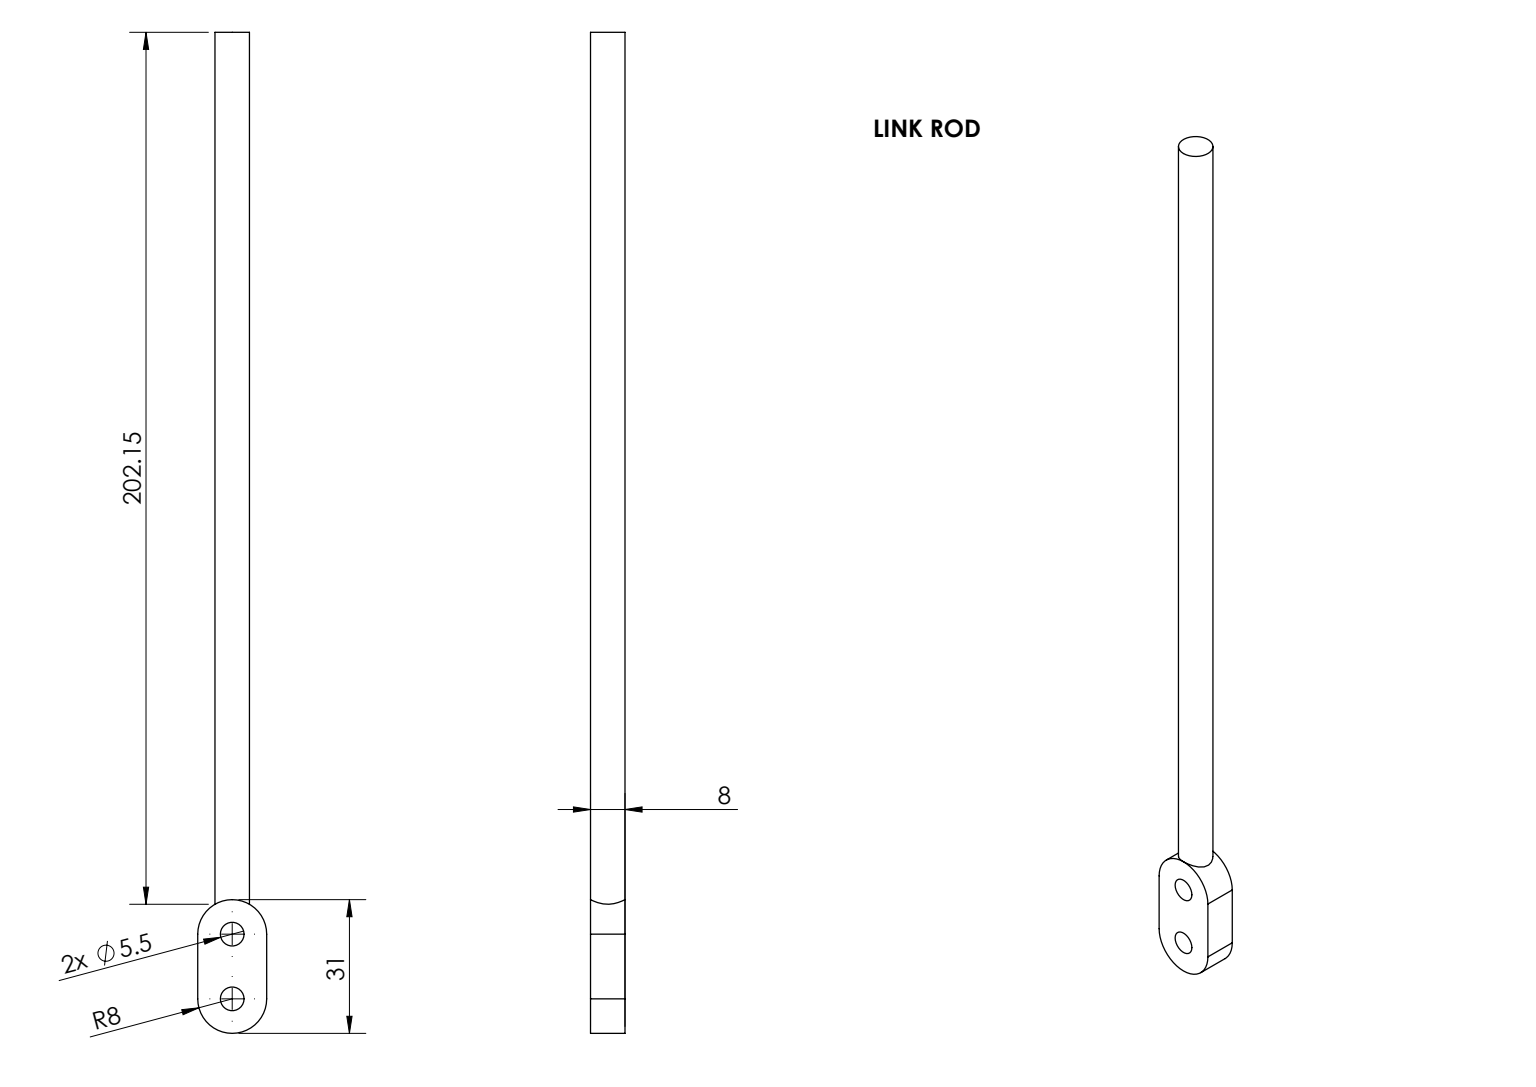
ISO-10303-21;
HEADER;
FILE_DESCRIPTION (('STEP AP214'),
    '1' );
FILE_NAME ('link rod.step',
    '2026-09-24T10:26:00',
    ( '' ),
    ( '' ),
    'SwSTEP 2.0',
    'SolidWorks 2026',
    '' );
FILE_SCHEMA (( 'AUTOMOTIVE_DESIGN' ));
ENDSEC;

DATA;
#140=DIRECTION ( 'NONE',  ( 0.000000000000000000, 1.000000000000000000, 0.000000000000000000 ) ) ;
#167=CARTESIAN_POINT ( 'NONE',  ( 0.000000000000000000, 0.000000000000000000, 0.000000000000000000 ) ) ;
#178=LINE ( 'NONE', #1338, #11397 ) ;
#188=AXIS2_PLACEMENT_3D ( 'NONE', #12778, #9636, #495 ) ;
#201=VECTOR ( 'NONE', #12349, 1000.000000000000000 ) ;
#214=CARTESIAN_POINT ( 'NONE',  ( 8.000000000000000000, 25.49999999999996803, 8.000000000000007105 ) ) ;
#231=FILL_AREA_STYLE_COLOUR ( '', #8450 ) ;
#235=CARTESIAN_POINT ( 'NONE',  ( 0.000000000000000000, 25.49999999999996803, 8.000000000000007105 ) ) ;
#292=ORIENTED_EDGE ( 'NONE', *, *, #11801, .F. ) ;
#308=AXIS2_PLACEMENT_3D ( 'NONE', #4405, #11111, #14418 ) ;
#313=VERTEX_POINT ( 'NONE', #3807 ) ;
#351=DIRECTION ( 'NONE',  ( 0.000000000000000000, 0.000000000000000000, 1.000000000000000000 ) ) ;
#354=CARTESIAN_POINT ( 'NONE',  ( -2.749999999999997780, 25.49999999999996803, 8.000000000000007105 ) ) ;
#363=FACE_BOUND ( 'NONE', #5930, .T. ) ;
#377=ADVANCED_FACE ( 'NONE', ( #4324 ), #12061, .F. ) ;
#423=VECTOR ( 'NONE', #878, 1000.000000000000000 ) ;
#495=DIRECTION ( 'NONE',  ( 1.000000000000000000, 0.000000000000000000, 0.000000000000000000 ) ) ;
#501=DIRECTION ( 'NONE',  ( 0.000000000000000000, 0.000000000000000000, -1.000000000000000000 ) ) ;
#504=EDGE_LOOP ( 'NONE', ( #9711, #6187, #8657, #5376, #2686 ) ) ;
#531=FACE_OUTER_BOUND ( 'NONE', #7015, .T. ) ;
#549=VERTEX_POINT ( 'NONE', #5876 ) ;
#557=ADVANCED_FACE ( 'NONE', ( #2536 ), #12548, .F. ) ;
#617=ORIENTED_EDGE ( 'NONE', *, *, #13492, .F. ) ;
#662=EDGE_CURVE ( 'NONE', #4679, #9332, #11674, .T. ) ;
#667=CARTESIAN_POINT ( 'NONE',  ( 2.450325270861126281, 48.11882021490242778, 7.172319002129951215 ) ) ;
#827=AXIS2_PLACEMENT_3D ( 'NONE', #1064, #4522, #2445 ) ;
#840=CARTESIAN_POINT ( 'NONE',  ( -3.010143253645307659, 47.91462539009204136, 1.353322078536347339 ) ) ;
#846=DIRECTION ( 'NONE',  ( 0.000000000000000000, 0.000000000000000000, 1.000000000000000000 ) ) ;
#859=CARTESIAN_POINT ( 'NONE',  ( 3.466359554492712824, 47.71176265719417131, 6.012830585829956220 ) ) ;
#878=DIRECTION ( 'NONE',  ( 0.000000000000000000, 1.000000000000000000, 0.000000000000000000 ) ) ;
#886=EDGE_CURVE ( 'NONE', #11486, #7236, #4159, .T. ) ;
#927=CARTESIAN_POINT ( 'NONE',  ( 3.973244831464914029, 47.44383994248515535, 3.467973375954350512 ) ) ;
#978=VECTOR ( 'NONE', #140, 1000.000000000000000 ) ;
#1006=LINE ( 'NONE', #1078, #7921 ) ;
#1010=LINE ( 'NONE', #4471, #7742 ) ;
#1036=EDGE_LOOP ( 'NONE', ( #12151, #2448, #6023, #13812 ) ) ;
#1048=CARTESIAN_POINT ( 'NONE',  ( 2.750000000000003553, 40.49999999999999289, 8.000000000000007105 ) ) ;
#1064=CARTESIAN_POINT ( 'NONE',  ( 0.000000000000000000, 40.49999999999999289, 8.000000000000007105 ) ) ;
#1078=CARTESIAN_POINT ( 'NONE',  ( -8.000000000000000000, 40.49999999999999289, 8.000000000000007105 ) ) ;
#1113=DIRECTION ( 'NONE',  ( 0.000000000000000000, 0.000000000000000000, 1.000000000000000000 ) ) ;
#1200=( GEOMETRIC_REPRESENTATION_CONTEXT ( 3 ) GLOBAL_UNCERTAINTY_ASSIGNED_CONTEXT ( ( #2815 ) ) GLOBAL_UNIT_ASSIGNED_CONTEXT ( ( #12457, #5770, #9006 ) ) REPRESENTATION_CONTEXT ( 'NONE', 'WORKASPACE' ) );
#1227=CARTESIAN_POINT ( 'NONE',  ( 0.000000000000000000, 17.49899999999995970, 4.000000000000003553 ) ) ;
#1240=CARTESIAN_POINT ( 'NONE',  ( -2.749999999999997780, 25.49999999999996803, 8.000000000000007105 ) ) ;
#1247=DIRECTION ( 'NONE',  ( 0.000000000000000000, 0.000000000000000000, 1.000000000000000000 ) ) ;
#1257=VERTEX_POINT ( 'NONE', #4208 ) ;
#1297=EDGE_CURVE ( 'NONE', #1257, #9332, #10297, .T. ) ;
#1338=CARTESIAN_POINT ( 'NONE',  ( 0.000000000000000000, 17.49899999999995970, 8.000000000000003553 ) ) ;
#1374=LINE ( 'NONE', #9204, #8230 ) ;
#1387=EDGE_CURVE ( 'NONE', #5595, #313, #12174, .T. ) ;
#1395=CYLINDRICAL_SURFACE ( 'NONE', #5325, 8.000000000000000000 ) ;
#1422=EDGE_LOOP ( 'NONE', ( #3931, #617 ) ) ;
#1441=CARTESIAN_POINT ( 'NONE',  ( 0.000000000000000000, 40.49999999999999289, 8.000000000000007105 ) ) ;
#1465=CIRCLE ( 'NONE', #308, 2.749999999999997780 ) ;
#1511=CARTESIAN_POINT ( 'NONE',  ( -2.450325270861127613, 48.11882021490243488, 7.172319002129952992 ) ) ;
#1547=ORIENTED_EDGE ( 'NONE', *, *, #6614, .T. ) ;
#1572=EDGE_LOOP ( 'NONE', ( #7051, #8246 ) ) ;
#1581=FACE_OUTER_BOUND ( 'NONE', #504, .T. ) ;
#1592=ORIENTED_EDGE ( 'NONE', *, *, #11567, .F. ) ;
#1613=FACE_OUTER_BOUND ( 'NONE', #5829, .T. ) ;
#1622=ADVANCED_FACE ( 'NONE', ( #7977 ), #11348, .T. ) ;
#1656=EDGE_LOOP ( 'NONE', ( #4322, #4081, #13598, #12074 ) ) ;
#1691=ADVANCED_FACE ( 'NONE', ( #13566 ), #3537, .F. ) ;
#1693=VERTEX_POINT ( 'NONE', #6222 ) ;
#1714=ORIENTED_EDGE ( 'NONE', *, *, #6615, .T. ) ;
#1724=DIRECTION ( 'NONE',  ( 0.000000000000000000, 0.000000000000000000, 1.000000000000000000 ) ) ;
#1757=CARTESIAN_POINT ( 'NONE',  ( 1.051966859446179514, 48.43488408057972805, 0.1316037626694079310 ) ) ;
#1770=CIRCLE ( 'NONE', #11106, 2.750000000000003553 ) ;
#1805=CARTESIAN_POINT ( 'NONE',  ( -3.466359554492713269, 47.71176265719419973, 6.012830585829961549 ) ) ;
#1825=ADVANCED_FACE ( 'NONE', ( #531 ), #9525, .T. ) ;
#1837=VECTOR ( 'NONE', #8930, 1000.000000000000000 ) ;
#1857=VERTEX_POINT ( 'NONE', #13124 ) ;
#1893=DIRECTION ( 'NONE',  ( 0.000000000000000000, 0.000000000000000000, -1.000000000000000000 ) ) ;
#1912=CIRCLE ( 'NONE', #11248, 8.000000000000000000 ) ;
#1969=ORIENTED_EDGE ( 'NONE', *, *, #4883, .F. ) ;
#1998=CARTESIAN_POINT ( 'NONE',  ( 0.000000000000000000, 48.49999999999999289, 0.000000000000000000 ) ) ;
#2053=DIRECTION ( 'NONE',  ( 0.000000000000000000, 0.000000000000000000, -1.000000000000000000 ) ) ;
#2106=CARTESIAN_POINT ( 'NONE',  ( 0.000000000000000000, 40.49999999999999289, 8.000000000000007105 ) ) ;
#2140=CARTESIAN_POINT ( 'NONE',  ( 8.000000000000000000, 25.49999999999996803, 0.000000000000000000 ) ) ;
#2148=FACE_OUTER_BOUND ( 'NONE', #13063, .T. ) ;
#2189=CARTESIAN_POINT ( 'NONE',  ( 0.000000000000000000, 249.5765550933606391, 8.000000000000003553 ) ) ;
#2229=EDGE_LOOP ( 'NONE', ( #1714, #13927, #11939, #1969 ) ) ;
#2260=DIRECTION ( 'NONE',  ( 0.000000000000000000, 0.000000000000000000, 1.000000000000000000 ) ) ;
#2284=EDGE_CURVE ( 'NONE', #6358, #9561, #1006, .T. ) ;
#2333=AXIS2_PLACEMENT_3D ( 'NONE', #14004, #2053, #4343 ) ;
#2411=EDGE_CURVE ( 'NONE', #6243, #549, #10151, .T. ) ;
#2426=VECTOR ( 'NONE', #5088, 1000.000000000000000 ) ;
#2430=SURFACE_SIDE_STYLE ('',( #5840 ) ) ;
#2445=DIRECTION ( 'NONE',  ( 1.000000000000000000, 0.000000000000000000, 0.000000000000000000 ) ) ;
#2448=ORIENTED_EDGE ( 'NONE', *, *, #6615, .F. ) ;
#2536=FACE_OUTER_BOUND ( 'NONE', #12567, .T. ) ;
#2583=ORIENTED_EDGE ( 'NONE', *, *, #2706, .T. ) ;
#2686=ORIENTED_EDGE ( 'NONE', *, *, #11415, .T. ) ;
#2706=EDGE_CURVE ( 'NONE', #4722, #12253, #4867, .T. ) ;
#2789=AXIS2_PLACEMENT_3D ( 'NONE', #8599, #3200, #3065 ) ;
#2791=CARTESIAN_POINT ( 'NONE',  ( 8.000000000000000000, 40.49999999999999289, 8.000000000000007105 ) ) ;
#2802=CIRCLE ( 'NONE', #9799, 2.750000000000003553 ) ;
#2815=UNCERTAINTY_MEASURE_WITH_UNIT (LENGTH_MEASURE( 1.000000000000000082E-05 ), #12457, 'distance_accuracy_value', 'NONE');
#2866=DIRECTION ( 'NONE',  ( 1.000000000000000000, 0.000000000000000000, 0.000000000000000000 ) ) ;
#2908=EDGE_CURVE ( 'NONE', #313, #5595, #8361, .T. ) ;
#2927=PRESENTATION_STYLE_ASSIGNMENT (( #10808 ) ) ;
#2941=CARTESIAN_POINT ( 'NONE',  ( 1.305984381679704098, 48.39647413643795204, 0.2102513847387766921 ) ) ;
#2988=CARTESIAN_POINT ( 'NONE',  ( -3.012791009409888865, 47.91354231080889292, 6.643648411893776640 ) ) ;
#2993=FILL_AREA_STYLE ('',( #6260 ) ) ;
#3013=CARTESIAN_POINT ( 'NONE',  ( 2.647226096189656985, 48.05180945724377750, 0.9903388192220060615 ) ) ;
#3018=CARTESIAN_POINT ( 'NONE',  ( 0.000000000000000000, 25.49999999999996803, 8.000000000000007105 ) ) ;
#3038=EDGE_LOOP ( 'NONE', ( #1547, #11800, #11167, #13440 ) ) ;
#3065=DIRECTION ( 'NONE',  ( 1.000000000000000000, 0.000000000000000000, 0.000000000000000000 ) ) ;
#3070=DIRECTION ( 'NONE',  ( 0.000000000000000000, 0.000000000000000000, 1.000000000000000000 ) ) ;
#3095=ADVANCED_FACE ( 'NONE', ( #13196 ), #7597, .T. ) ;
#3152=CARTESIAN_POINT ( 'NONE',  ( 3.973178806327566370, 47.44387873568884118, 4.532639216498019152 ) ) ;
#3178=CARTESIAN_POINT ( 'NONE',  ( 8.000000000000000000, 25.49999999999996803, 8.000000000000007105 ) ) ;
#3200=DIRECTION ( 'NONE',  ( 0.000000000000000000, 0.000000000000000000, 1.000000000000000000 ) ) ;
#3216=CARTESIAN_POINT ( 'NONE',  ( 3.010143253645308992, 47.91462539009204136, 1.353322078536349338 ) ) ;
#3249=PLANE ( 'NONE',  #7377 ) ;
#3405=SURFACE_STYLE_USAGE ( .BOTH. , #2430 ) ;
#3427=CARTESIAN_POINT ( 'NONE',  ( 0.000000000000000000, 40.49999999999999289, 8.000000000000007105 ) ) ;
#3451=DIRECTION ( 'NONE',  ( 0.000000000000000000, 1.000000000000000000, 0.000000000000000000 ) ) ;
#3511=CARTESIAN_POINT ( 'NONE',  ( 4.898587196589412829E-16, 17.49899999999995970, 3.469446951953614189E-15 ) ) ;
#3530=EDGE_CURVE ( 'NONE', #1693, #14098, #3551, .T. ) ;
#3537=CYLINDRICAL_SURFACE ( 'NONE', #11716, 2.749999999999997780 ) ;
#3540=PRESENTATION_STYLE_ASSIGNMENT (( #3405 ) ) ;
#3551=B_SPLINE_CURVE_WITH_KNOTS ( 'NONE', 3,
 ( #4803, #10508, #12855, #5877, #10363, #12619, #13741, #1511, #5953, #2988, #13224, #1805, #13015, #10935, #9563, #5167, #13159, #7486, #14113, #5304, #14041, #4008, #8595, #5240, #840, #8456, #9705, #5375, #8671, #9767, #7419, #4308, #4097, #6400 ),
 .UNSPECIFIED., .F., .F.,
 ( 4, 2, 2, 2, 2, 2, 2, 2, 2, 2, 2, 2, 2, 2, 2, 2, 4 ),
 ( 0.000000000000000000, 0.0007952457144059360810, 0.001590491428811872162, 0.002385737143217809327, 0.003180982857623746492, 0.003976228572029682357, 0.004771474286435620389, 0.005566720000841557554, 0.006361965715247495587, 0.007157211429653434487, 0.007952457144059371652, 0.008747702858465312287, 0.009542948572871249452, 0.01033819428727718835, 0.01113344000168312725, 0.01192868571608906615, 0.01272393143049500505 ),
 .UNSPECIFIED. ) ;
#3584=LINE ( 'NONE', #9339, #7245 ) ;
#3610=( NAMED_UNIT ( * ) PLANE_ANGLE_UNIT ( ) SI_UNIT ( $, .RADIAN. ) );
#3633=FACE_OUTER_BOUND ( 'NONE', #6702, .T. ) ;
#3649=CYLINDRICAL_SURFACE ( 'NONE', #12102, 4.000000000000000000 ) ;
#3656=PRODUCT_DEFINITION ( 'UNKNOWN', '', #8021, #10108 ) ;
#3720=( GEOMETRIC_REPRESENTATION_CONTEXT ( 3 ) GLOBAL_UNCERTAINTY_ASSIGNED_CONTEXT ( ( #6001 ) ) GLOBAL_UNIT_ASSIGNED_CONTEXT ( ( #13961, #3939, #6335 ) ) REPRESENTATION_CONTEXT ( 'NONE', 'WORKASPACE' ) );
#3807=CARTESIAN_POINT ( 'NONE',  ( 4.898587196589412829E-16, 249.5765550933606391, 3.469446951953614189E-15 ) ) ;
#3931=ORIENTED_EDGE ( 'NONE', *, *, #2706, .F. ) ;
#3939=( NAMED_UNIT ( * ) PLANE_ANGLE_UNIT ( ) SI_UNIT ( $, .RADIAN. ) );
#4008=CARTESIAN_POINT ( 'NONE',  ( -3.587774770580208550, 47.65128983029578080, 2.212041269487583950 ) ) ;
#4074=ADVANCED_FACE ( 'NONE', ( #2148 ), #3249, .F. ) ;
#4081=ORIENTED_EDGE ( 'NONE', *, *, #3530, .T. ) ;
#4088=DIRECTION ( 'NONE',  ( 0.000000000000000000, 0.000000000000000000, 1.000000000000000000 ) ) ;
#4097=CARTESIAN_POINT ( 'NONE',  ( -0.2655919857739738044, 48.49999999999998579, 9.914050073752000185E-16 ) ) ;
#4118=CARTESIAN_POINT ( 'NONE',  ( 0.000000000000000000, 25.49999999999996803, 0.000000000000000000 ) ) ;
#4119=DIRECTION ( 'NONE',  ( 1.000000000000000000, 0.000000000000000000, 0.000000000000000000 ) ) ;
#4159=LINE ( 'NONE', #9704, #8506 ) ;
#4171=DIRECTION ( 'NONE',  ( 1.000000000000000000, 0.000000000000000000, 0.000000000000000000 ) ) ;
#4180=CARTESIAN_POINT ( 'NONE',  ( 3.176101805495866071, 47.84421704054535240, 1.554735638783587337 ) ) ;
#4208=CARTESIAN_POINT ( 'NONE',  ( -8.000000000000000000, 25.49999999999996803, 0.000000000000000000 ) ) ;
#4222=CIRCLE ( 'NONE', #7930, 2.749999999999997780 ) ;
#4224=DIRECTION ( 'NONE',  ( 1.000000000000000000, 0.000000000000000000, 0.000000000000000000 ) ) ;
#4226=ORIENTED_EDGE ( 'NONE', *, *, #8091, .T. ) ;
#4269=STYLED_ITEM ( 'NONE', ( #3540 ), #11166 ) ;
#4308=CARTESIAN_POINT ( 'NONE',  ( -0.5291067203508891259, 48.48680572720347470, 0.02618951120639553473 ) ) ;
#4322=ORIENTED_EDGE ( 'NONE', *, *, #4979, .F. ) ;
#4324=FACE_OUTER_BOUND ( 'NONE', #3038, .T. ) ;
#4330=CARTESIAN_POINT ( 'NONE',  ( -2.750000000000003553, 40.49999999999999289, 8.000000000000007105 ) ) ;
#4333=ADVANCED_FACE ( 'NONE', ( #1613 ), #13925, .F. ) ;
#4343=DIRECTION ( 'NONE',  ( -1.000000000000000000, 0.000000000000000000, 0.000000000000000000 ) ) ;
#4381=ORIENTED_EDGE ( 'NONE', *, *, #12499, .T. ) ;
#4405=CARTESIAN_POINT ( 'NONE',  ( 0.000000000000000000, 25.49999999999996803, 8.000000000000007105 ) ) ;
#4432=SHAPE_REPRESENTATION ( 'link rod', ( #11025 ), #1200 ) ;
#4453=DIRECTION ( 'NONE',  ( 1.000000000000000000, 0.000000000000000000, 0.000000000000000000 ) ) ;
#4471=CARTESIAN_POINT ( 'NONE',  ( -8.000000000000000000, 25.49999999999996803, 8.000000000000007105 ) ) ;
#4522=DIRECTION ( 'NONE',  ( 0.000000000000000000, 0.000000000000000000, 1.000000000000000000 ) ) ;
#4575=DIRECTION ( 'NONE',  ( 0.000000000000000000, 0.000000000000000000, -1.000000000000000000 ) ) ;
#4580=DIRECTION ( 'NONE',  ( 0.000000000000000000, 0.000000000000000000, 1.000000000000000000 ) ) ;
#4595=ORIENTED_EDGE ( 'NONE', *, *, #7703, .F. ) ;
#4630=EDGE_CURVE ( 'NONE', #4679, #1857, #1374, .T. ) ;
#4679=VERTEX_POINT ( 'NONE', #214 ) ;
#4722=VERTEX_POINT ( 'NONE', #1240 ) ;
#4777=CARTESIAN_POINT ( 'NONE',  ( 0.000000000000000000, 40.49999999999999289, 8.000000000000007105 ) ) ;
#4795=ORIENTED_EDGE ( 'NONE', *, *, #5526, .T. ) ;
#4803=CARTESIAN_POINT ( 'NONE',  ( 0.000000000000000000, 48.49999999999999289, 8.000000000000007105 ) ) ;
#4819=DIRECTION ( 'NONE',  ( 0.000000000000000000, 1.000000000000000000, 0.000000000000000000 ) ) ;
#4865=AXIS2_PLACEMENT_3D ( 'NONE', #13089, #846, #13164 ) ;
#4867=CIRCLE ( 'NONE', #2789, 2.749999999999997780 ) ;
#4883=EDGE_CURVE ( 'NONE', #1693, #5595, #178, .T. ) ;
#4979=EDGE_CURVE ( 'NONE', #1693, #6358, #14391, .T. ) ;
#4991=EDGE_CURVE ( 'NONE', #549, #7236, #1770, .T. ) ;
#5012=DIRECTION ( 'NONE',  ( 0.000000000000000000, 0.000000000000000000, 1.000000000000000000 ) ) ;
#5049=FACE_OUTER_BOUND ( 'NONE', #10526, .T. ) ;
#5088=DIRECTION ( 'NONE',  ( 0.000000000000000000, 0.000000000000000000, -1.000000000000000000 ) ) ;
#5114=DIRECTION ( 'NONE',  ( -1.000000000000000000, 0.000000000000000000, 0.000000000000000000 ) ) ;
#5167=CARTESIAN_POINT ( 'NONE',  ( -3.973178806327567258, 47.44387873568886249, 4.532639216498020929 ) ) ;
#5188=CARTESIAN_POINT ( 'NONE',  ( 0.5330603548786414514, 48.48645934998781115, 7.973110123615591682 ) ) ;
#5240=CARTESIAN_POINT ( 'NONE',  ( -3.176101805495866515, 47.84421704054533819, 1.554735638783587337 ) ) ;
#5260=VERTEX_POINT ( 'NONE', #9822 ) ;
#5261=CARTESIAN_POINT ( 'NONE',  ( 0.000000000000000000, 25.49999999999996803, 0.000000000000000000 ) ) ;
#5304=CARTESIAN_POINT ( 'NONE',  ( -3.868826622783372304, 47.50255440539073959, 2.950282236837605154 ) ) ;
#5316=ADVANCED_FACE ( 'NONE', ( #12569, #363, #7143 ), #13837, .F. ) ;
#5325=AXIS2_PLACEMENT_3D ( 'NONE', #4777, #9229, #13712 ) ;
#5375=CARTESIAN_POINT ( 'NONE',  ( -2.015657056808819014, 48.24519377879725113, 0.5351343119442694141 ) ) ;
#5376=ORIENTED_EDGE ( 'NONE', *, *, #4979, .T. ) ;
#5441=DIRECTION ( 'NONE',  ( 1.000000000000000000, 0.000000000000000000, 0.000000000000000000 ) ) ;
#5526=EDGE_CURVE ( 'NONE', #9673, #5260, #4222, .T. ) ;
#5534=DIRECTION ( 'NONE',  ( 0.000000000000000000, 0.000000000000000000, -1.000000000000000000 ) ) ;
#5540=CIRCLE ( 'NONE', #6935, 8.000000000000000000 ) ;
#5560=LINE ( 'NONE', #2140, #423 ) ;
#5595=VERTEX_POINT ( 'NONE', #2189 ) ;
#5644=ORIENTED_EDGE ( 'NONE', *, *, #662, .F. ) ;
#5648=PRODUCT ( 'link rod', 'link rod', '', ( #11929 ) ) ;
#5669=VERTEX_POINT ( 'NONE', #11243 ) ;
#5770=( NAMED_UNIT ( * ) PLANE_ANGLE_UNIT ( ) SI_UNIT ( $, .RADIAN. ) );
#5776=DIRECTION ( 'NONE',  ( 1.000000000000000000, 0.000000000000000000, 0.000000000000000000 ) ) ;
#5780=COLOUR_RGB ( '', 0.08235294, 0.09019608, 0.10196078) ;
#5829=EDGE_LOOP ( 'NONE', ( #11775, #10763, #8742, #10420 ) ) ;
#5835=AXIS2_PLACEMENT_3D ( 'NONE', #11593, #9253, #6100 ) ;
#5840=SURFACE_STYLE_FILL_AREA ( #13567 ) ;
#5876=CARTESIAN_POINT ( 'NONE',  ( 2.750000000000003553, 40.49999999999999289, 0.000000000000000000 ) ) ;
#5877=CARTESIAN_POINT ( 'NONE',  ( -1.050836307075461606, 48.43494986415684878, 7.868526909826536020 ) ) ;
#5920=CARTESIAN_POINT ( 'NONE',  ( 0.000000000000000000, 40.49999999999999289, 8.000000000000007105 ) ) ;
#5930=EDGE_LOOP ( 'NONE', ( #4795, #6999 ) ) ;
#5953=CARTESIAN_POINT ( 'NONE',  ( -2.650472254991408150, 48.05066328782152851, 7.006789553262803949 ) ) ;
#5971=DIRECTION ( 'NONE',  ( 1.000000000000000000, 0.000000000000000000, 0.000000000000000000 ) ) ;
#6001=UNCERTAINTY_MEASURE_WITH_UNIT (LENGTH_MEASURE( 1.000000000000000082E-05 ), #13961, 'distance_accuracy_value', 'NONE');
#6017=CIRCLE ( 'NONE', #7902, 2.750000000000003553 ) ;
#6023=ORIENTED_EDGE ( 'NONE', *, *, #11542, .F. ) ;
#6053=DIRECTION ( 'NONE',  ( 0.000000000000000000, 0.000000000000000000, 1.000000000000000000 ) ) ;
#6058=AXIS2_PLACEMENT_3D ( 'NONE', #11550, #11400, #5971 ) ;
#6100=DIRECTION ( 'NONE',  ( 0.000000000000000000, 0.000000000000000000, 1.000000000000000000 ) ) ;
#6133=ORIENTED_EDGE ( 'NONE', *, *, #2908, .F. ) ;
#6134=CARTESIAN_POINT ( 'NONE',  ( 0.000000000000000000, 40.49999999999999289, 0.000000000000000000 ) ) ;
#6187=ORIENTED_EDGE ( 'NONE', *, *, #4630, .T. ) ;
#6210=CARTESIAN_POINT ( 'NONE',  ( 0.5291067203508894590, 48.48680572720346049, 0.02618951120639558677 ) ) ;
#6222=CARTESIAN_POINT ( 'NONE',  ( 0.000000000000000000, 48.49999999999999289, 8.000000000000007105 ) ) ;
#6243=VERTEX_POINT ( 'NONE', #1048 ) ;
#6260=FILL_AREA_STYLE_COLOUR ( '', #5780 ) ;
#6332=AXIS2_PLACEMENT_3D ( 'NONE', #14091, #9818, #8723 ) ;
#6335=( NAMED_UNIT ( * ) SI_UNIT ( $, .STERADIAN. ) SOLID_ANGLE_UNIT ( ) );
#6350=CARTESIAN_POINT ( 'NONE',  ( 0.2655919857739733603, 48.49999999999999289, 9.644881826068967185E-16 ) ) ;
#6358=VERTEX_POINT ( 'NONE', #13208 ) ;
#6400=CARTESIAN_POINT ( 'NONE',  ( 0.000000000000000000, 48.49999999999999289, 0.000000000000000000 ) ) ;
#6419=CARTESIAN_POINT ( 'NONE',  ( 0.000000000000000000, 40.49999999999999289, 8.000000000000007105 ) ) ;
#6466=B_SPLINE_CURVE_WITH_KNOTS ( 'NONE', 3,
 ( #8551, #6482, #5188, #9789, #10889, #8483, #11783, #667, #14339, #9723, #14267, #859, #13032, #8694, #11926, #3152, #10958, #7582, #927, #14198, #9655, #8623, #11852, #4180, #3216, #3013, #8762, #7443, #13241, #2941, #1757, #6210, #6350, #10680 ),
 .UNSPECIFIED., .F., .F.,
 ( 4, 2, 2, 2, 2, 2, 2, 2, 2, 2, 2, 2, 2, 2, 2, 2, 4 ),
 ( 0.000000000000000000, 0.0007952457144059375989, 0.001590491428811875198, 0.002385737143217811929, 0.003180982857623748661, 0.003976228572029685826, 0.004771474286435622991, 0.005566720000841560156, 0.006361965715247496454, 0.007157211429653435354, 0.007952457144059375121, 0.008747702858465312287, 0.009542948572871252921, 0.01033819428727719182, 0.01113344000168312899, 0.01192868571608906962, 0.01272393143049500679 ),
 .UNSPECIFIED. ) ;
#6482=CARTESIAN_POINT ( 'NONE',  ( 0.2691907178497377484, 48.49999999999999289, 8.000000000000008882 ) ) ;
#6524=DIRECTION ( 'NONE',  ( 0.000000000000000000, 0.000000000000000000, 1.000000000000000000 ) ) ;
#6614=EDGE_CURVE ( 'NONE', #11486, #6243, #2802, .T. ) ;
#6615=EDGE_CURVE ( 'NONE', #1693, #14098, #6466, .T. ) ;
#6641=CLOSED_SHELL ( 'NONE', ( #3095, #377, #1691, #1622, #9393, #5316, #1825, #4074, #7709, #4333, #10182, #557, #9207, #7256 ) ) ;
#6687=DIRECTION ( 'NONE',  ( 0.000000000000000000, 1.000000000000000000, 0.000000000000000000 ) ) ;
#6702=EDGE_LOOP ( 'NONE', ( #11336, #13291 ) ) ;
#6717=ORIENTED_EDGE ( 'NONE', *, *, #11567, .T. ) ;
#6807=CARTESIAN_POINT ( 'NONE',  ( -8.000000000000000000, 25.49999999999996803, 8.000000000000007105 ) ) ;
#6826=VERTEX_POINT ( 'NONE', #6916 ) ;
#6873=MANIFOLD_SOLID_BREP ( 'Boss-Extrude2', #6641 ) ;
#6902=LINE ( 'NONE', #11368, #13132 ) ;
#6903=ORIENTED_EDGE ( 'NONE', *, *, #10923, .F. ) ;
#6916=CARTESIAN_POINT ( 'NONE',  ( -8.000000000000000000, 25.49999999999996803, 8.000000000000007105 ) ) ;
#6935=AXIS2_PLACEMENT_3D ( 'NONE', #9481, #4088, #4224 ) ;
#6999=ORIENTED_EDGE ( 'NONE', *, *, #10923, .T. ) ;
#7015=EDGE_LOOP ( 'NONE', ( #8069, #5644, #4595, #4226 ) ) ;
#7051=ORIENTED_EDGE ( 'NONE', *, *, #8195, .T. ) ;
#7067=APPLICATION_CONTEXT ( 'automotive_design' ) ;
#7139=LINE ( 'NONE', #6807, #1837 ) ;
#7143=FACE_BOUND ( 'NONE', #1572, .T. ) ;
#7198=CIRCLE ( 'NONE', #4865, 2.750000000000003553 ) ;
#7227=DIRECTION ( 'NONE',  ( 0.000000000000000000, 0.000000000000000000, -1.000000000000000000 ) ) ;
#7231=CARTESIAN_POINT ( 'NONE',  ( 2.749999999999997780, 25.49999999999996803, 8.000000000000007105 ) ) ;
#7236=VERTEX_POINT ( 'NONE', #8216 ) ;
#7245=VECTOR ( 'NONE', #13826, 1000.000000000000000 ) ;
#7256=ADVANCED_FACE ( 'NONE', ( #3633 ), #8067, .T. ) ;
#7288=SURFACE_SIDE_STYLE ('',( #10735 ) ) ;
#7290=FACE_BOUND ( 'NONE', #9103, .T. ) ;
#7312=CYLINDRICAL_SURFACE ( 'NONE', #10558, 2.749999999999997780 ) ;
#7377=AXIS2_PLACEMENT_3D ( 'NONE', #3178, #9819, #1113 ) ;
#7419=CARTESIAN_POINT ( 'NONE',  ( -1.051966859446179292, 48.43488408057972805, 0.1316037626694079032 ) ) ;
#7443=CARTESIAN_POINT ( 'NONE',  ( 2.015657056808820791, 48.24519377879725113, 0.5351343119442704133 ) ) ;
#7455=DIRECTION ( 'NONE',  ( 0.000000000000000000, 0.000000000000000000, -1.000000000000000000 ) ) ;
#7473=DIRECTION ( 'NONE',  ( 0.000000000000000000, 1.000000000000000000, 0.000000000000000000 ) ) ;
#7486=CARTESIAN_POINT ( 'NONE',  ( -4.000255272253210315, 47.42805584886342274, 3.737655343436113942 ) ) ;
#7511=DIRECTION ( 'NONE',  ( 0.000000000000000000, 0.000000000000000000, 1.000000000000000000 ) ) ;
#7533=AXIS2_PLACEMENT_3D ( 'NONE', #9594, #9737, #13046 ) ;
#7582=CARTESIAN_POINT ( 'NONE',  ( 4.000255272253209426, 47.42805584886342274, 3.737655343436113498 ) ) ;
#7597=CYLINDRICAL_SURFACE ( 'NONE', #10192, 4.000000000000000000 ) ;
#7703=EDGE_CURVE ( 'NONE', #6826, #4679, #10005, .T. ) ;
#7709=ADVANCED_FACE ( 'NONE', ( #12521 ), #1395, .T. ) ;
#7742=VECTOR ( 'NONE', #13313, 1000.000000000000000 ) ;
#7802=DIRECTION ( 'NONE',  ( -1.000000000000000000, 0.000000000000000000, 0.000000000000000000 ) ) ;
#7840=( NAMED_UNIT ( * ) SI_UNIT ( $, .STERADIAN. ) SOLID_ANGLE_UNIT ( ) );
#7842=ORIENTED_EDGE ( 'NONE', *, *, #4630, .F. ) ;
#7857=CARTESIAN_POINT ( 'NONE',  ( -2.749999999999997780, 25.49999999999996803, 0.000000000000000000 ) ) ;
#7869=EDGE_CURVE ( 'NONE', #9332, #5669, #5560, .T. ) ;
#7902=AXIS2_PLACEMENT_3D ( 'NONE', #8542, #3070, #4171 ) ;
#7921=VECTOR ( 'NONE', #5534, 1000.000000000000000 ) ;
#7930=AXIS2_PLACEMENT_3D ( 'NONE', #5261, #14265, #13977 ) ;
#7977=FACE_OUTER_BOUND ( 'NONE', #1656, .T. ) ;
#8021=PRODUCT_DEFINITION_FORMATION_WITH_SPECIFIED_SOURCE ( 'ANY', '', #5648, .NOT_KNOWN. ) ;
#8026=ORIENTED_EDGE ( 'NONE', *, *, #662, .T. ) ;
#8067=PLANE ( 'NONE',  #11389 ) ;
#8069=ORIENTED_EDGE ( 'NONE', *, *, #1297, .T. ) ;
#8089=APPLICATION_CONTEXT ( 'automotive_design' ) ;
#8091=EDGE_CURVE ( 'NONE', #6826, #1257, #7139, .T. ) ;
#8195=EDGE_CURVE ( 'NONE', #7236, #549, #6017, .T. ) ;
#8216=CARTESIAN_POINT ( 'NONE',  ( -2.750000000000003553, 40.49999999999999289, 0.000000000000000000 ) ) ;
#8230=VECTOR ( 'NONE', #4819, 1000.000000000000000 ) ;
#8235=CARTESIAN_POINT ( 'NONE',  ( 8.000000000000000000, 25.49999999999996803, 0.000000000000000000 ) ) ;
#8246=ORIENTED_EDGE ( 'NONE', *, *, #4991, .T. ) ;
#8271=ORIENTED_EDGE ( 'NONE', *, *, #11035, .F. ) ;
#8320=LINE ( 'NONE', #2791, #13370 ) ;
#8361=CIRCLE ( 'NONE', #10234, 4.000000000000000000 ) ;
#8450=COLOUR_RGB ( '', 0.08235294, 0.09019608, 0.10196078) ;
#8456=CARTESIAN_POINT ( 'NONE',  ( -2.647226096189655209, 48.05180945724376329, 0.9903388192220039521 ) ) ;
#8483=CARTESIAN_POINT ( 'NONE',  ( 1.790396195872467677, 48.30096731618027661, 7.586517658982192103 ) ) ;
#8506=VECTOR ( 'NONE', #11977, 1000.000000000000000 ) ;
#8517=EDGE_CURVE ( 'NONE', #5669, #14098, #5540, .T. ) ;
#8542=CARTESIAN_POINT ( 'NONE',  ( 0.000000000000000000, 40.49999999999999289, 0.000000000000000000 ) ) ;
#8551=CARTESIAN_POINT ( 'NONE',  ( 0.000000000000000000, 48.49999999999999289, 8.000000000000007105 ) ) ;
#8595=CARTESIAN_POINT ( 'NONE',  ( -3.464648251117637301, 47.71258338693829160, 1.984273587230471314 ) ) ;
#8599=CARTESIAN_POINT ( 'NONE',  ( 0.000000000000000000, 25.49999999999996803, 8.000000000000007105 ) ) ;
#8623=CARTESIAN_POINT ( 'NONE',  ( 3.587774770580208106, 47.65128983029576659, 2.212041269487582618 ) ) ;
#8657=ORIENTED_EDGE ( 'NONE', *, *, #11542, .T. ) ;
#8671=CARTESIAN_POINT ( 'NONE',  ( -1.786241414228626923, 48.30187417244851389, 0.4115279878254325396 ) ) ;
#8694=CARTESIAN_POINT ( 'NONE',  ( 3.789464654225618734, 47.54647181849109927, 5.306690203119769578 ) ) ;
#8723=DIRECTION ( 'NONE',  ( 1.000000000000000000, 0.000000000000000000, 0.000000000000000000 ) ) ;
#8742=ORIENTED_EDGE ( 'NONE', *, *, #11415, .F. ) ;
#8762=CARTESIAN_POINT ( 'NONE',  ( 2.448955312130046913, 48.11928591936100474, 0.8265499080465862347 ) ) ;
#8807=ORIENTED_EDGE ( 'NONE', *, *, #4991, .F. ) ;
#8900=CARTESIAN_POINT ( 'NONE',  ( 2.750000000000003553, 40.49999999999999289, 8.000000000000007105 ) ) ;
#8930=DIRECTION ( 'NONE',  ( 0.000000000000000000, 0.000000000000000000, -1.000000000000000000 ) ) ;
#8977=DIRECTION ( 'NONE',  ( 0.000000000000000000, 1.000000000000000000, 0.000000000000000000 ) ) ;
#9006=( NAMED_UNIT ( * ) SI_UNIT ( $, .STERADIAN. ) SOLID_ANGLE_UNIT ( ) );
#9065=ORIENTED_EDGE ( 'NONE', *, *, #11241, .F. ) ;
#9103=EDGE_LOOP ( 'NONE', ( #11846, #13625 ) ) ;
#9124=CIRCLE ( 'NONE', #12181, 2.749999999999997780 ) ;
#9204=CARTESIAN_POINT ( 'NONE',  ( 8.000000000000000000, 25.49999999999996803, 8.000000000000007105 ) ) ;
#9207=ADVANCED_FACE ( 'NONE', ( #9263 ), #3649, .T. ) ;
#9216=ORIENTED_EDGE ( 'NONE', *, *, #3530, .F. ) ;
#9229=DIRECTION ( 'NONE',  ( 0.000000000000000000, 0.000000000000000000, -1.000000000000000000 ) ) ;
#9253=DIRECTION ( 'NONE',  ( 0.000000000000000000, 1.000000000000000000, 0.000000000000000000 ) ) ;
#9263=FACE_OUTER_BOUND ( 'NONE', #10121, .T. ) ;
#9332=VERTEX_POINT ( 'NONE', #8235 ) ;
#9339=CARTESIAN_POINT ( 'NONE',  ( 2.749999999999997780, 25.49999999999996803, 8.000000000000007105 ) ) ;
#9371=DIRECTION ( 'NONE',  ( -1.000000000000000000, 0.000000000000000000, 0.000000000000000000 ) ) ;
#9375=( GEOMETRIC_REPRESENTATION_CONTEXT ( 3 ) GLOBAL_UNCERTAINTY_ASSIGNED_CONTEXT ( ( #13792 ) ) GLOBAL_UNIT_ASSIGNED_CONTEXT ( ( #10331, #3610, #7840 ) ) REPRESENTATION_CONTEXT ( 'NONE', 'WORKASPACE' ) );
#9393=ADVANCED_FACE ( 'NONE', ( #13897, #1581, #7290 ), #11837, .T. ) ;
#9460=EDGE_CURVE ( 'NONE', #6243, #11486, #7198, .T. ) ;
#9481=CARTESIAN_POINT ( 'NONE',  ( 0.000000000000000000, 40.49999999999999289, 0.000000000000000000 ) ) ;
#9525=CYLINDRICAL_SURFACE ( 'NONE', #2333, 8.000000000000000000 ) ;
#9560=EDGE_LOOP ( 'NONE', ( #13702, #292, #9065, #14057, #14058 ) ) ;
#9561=VERTEX_POINT ( 'NONE', #12267 ) ;
#9563=CARTESIAN_POINT ( 'NONE',  ( -3.868554393999076968, 47.50270580730570202, 5.050781263000355459 ) ) ;
#9594=CARTESIAN_POINT ( 'NONE',  ( -8.000000000000000000, 25.49999999999996803, 8.000000000000007105 ) ) ;
#9636=DIRECTION ( 'NONE',  ( 0.000000000000000000, 0.000000000000000000, 1.000000000000000000 ) ) ;
#9655=CARTESIAN_POINT ( 'NONE',  ( 3.790690275325682812, 47.54583148236281431, 2.696316195168958263 ) ) ;
#9673=VERTEX_POINT ( 'NONE', #7857 ) ;
#9704=CARTESIAN_POINT ( 'NONE',  ( -2.750000000000003553, 40.49999999999999289, 8.000000000000007105 ) ) ;
#9705=CARTESIAN_POINT ( 'NONE',  ( -2.448955312130046469, 48.11928591936100474, 0.8265499080465856796 ) ) ;
#9711=ORIENTED_EDGE ( 'NONE', *, *, #7703, .T. ) ;
#9723=CARTESIAN_POINT ( 'NONE',  ( 3.012791009409891085, 47.91354231080892134, 6.643648411893779304 ) ) ;
#9734=ORIENTED_EDGE ( 'NONE', *, *, #12499, .F. ) ;
#9737=DIRECTION ( 'NONE',  ( 1.000000000000000000, 0.000000000000000000, 0.000000000000000000 ) ) ;
#9767=CARTESIAN_POINT ( 'NONE',  ( -1.305984381679703654, 48.39647413643795915, 0.2102513847387771917 ) ) ;
#9789=CARTESIAN_POINT ( 'NONE',  ( 1.050836307075463827, 48.43494986415684167, 7.868526909826528914 ) ) ;
#9799=AXIS2_PLACEMENT_3D ( 'NONE', #6419, #7511, #9871 ) ;
#9818=DIRECTION ( 'NONE',  ( 0.000000000000000000, 0.000000000000000000, 1.000000000000000000 ) ) ;
#9819=DIRECTION ( 'NONE',  ( -1.000000000000000000, 0.000000000000000000, 0.000000000000000000 ) ) ;
#9822=CARTESIAN_POINT ( 'NONE',  ( 2.749999999999997780, 25.49999999999996803, 0.000000000000000000 ) ) ;
#9871=DIRECTION ( 'NONE',  ( 1.000000000000000000, 0.000000000000000000, 0.000000000000000000 ) ) ;
#9992=CARTESIAN_POINT ( 'NONE',  ( 0.000000000000000000, 40.49999999999999289, 0.000000000000000000 ) ) ;
#10005=CIRCLE ( 'NONE', #14454, 8.000000000000000000 ) ;
#10015=STYLED_ITEM ( 'NONE', ( #2927 ), #6873 ) ;
#10108=PRODUCT_DEFINITION_CONTEXT ( 'detailed design', #8089, 'design' ) ;
#10121=EDGE_LOOP ( 'NONE', ( #13710, #9216, #11437, #6133 ) ) ;
#10151=LINE ( 'NONE', #8900, #201 ) ;
#10168=CARTESIAN_POINT ( 'NONE',  ( 0.000000000000000000, 17.49899999999995970, 4.000000000000003553 ) ) ;
#10182=ADVANCED_FACE ( 'NONE', ( #5049 ), #7312, .F. ) ;
#10192=AXIS2_PLACEMENT_3D ( 'NONE', #10168, #3451, #1247 ) ;
#10222=LINE ( 'NONE', #354, #10798 ) ;
#10234=AXIS2_PLACEMENT_3D ( 'NONE', #11742, #11512, #5012 ) ;
#10297=CIRCLE ( 'NONE', #6332, 8.000000000000000000 ) ;
#10331=( LENGTH_UNIT ( ) NAMED_UNIT ( * ) SI_UNIT ( .MILLI., .METRE. ) );
#10363=CARTESIAN_POINT ( 'NONE',  ( -1.307332176164476278, 48.39629610561008377, 7.789394415675250372 ) ) ;
#10366=AXIS2_PLACEMENT_3D ( 'NONE', #2106, #1893, #10953 ) ;
#10420=ORIENTED_EDGE ( 'NONE', *, *, #2284, .T. ) ;
#10458=PRODUCT_DEFINITION_SHAPE ( 'NONE', 'NONE',  #3656 ) ;
#10508=CARTESIAN_POINT ( 'NONE',  ( -0.2691907178497369713, 48.50000000000000711, 8.000000000000007105 ) ) ;
#10526=EDGE_LOOP ( 'NONE', ( #1592, #12790, #4381, #6903 ) ) ;
#10558=AXIS2_PLACEMENT_3D ( 'NONE', #3018, #11857, #5114 ) ;
#10680=CARTESIAN_POINT ( 'NONE',  ( 0.000000000000000000, 48.49999999999999289, 0.000000000000000000 ) ) ;
#10735=SURFACE_STYLE_FILL_AREA ( #2993 ) ;
#10763=ORIENTED_EDGE ( 'NONE', *, *, #8091, .F. ) ;
#10798=VECTOR ( 'NONE', #501, 1000.000000000000000 ) ;
#10808=SURFACE_STYLE_USAGE ( .BOTH. , #7288 ) ;
#10889=CARTESIAN_POINT ( 'NONE',  ( 1.307332176164478943, 48.39629610561006956, 7.789394415675249483 ) ) ;
#10923=EDGE_CURVE ( 'NONE', #5260, #9673, #9124, .T. ) ;
#10935=CARTESIAN_POINT ( 'NONE',  ( -3.789464654225616513, 47.54647181849109217, 5.306690203119769578 ) ) ;
#10953=DIRECTION ( 'NONE',  ( -1.000000000000000000, 0.000000000000000000, 0.000000000000000000 ) ) ;
#10958=CARTESIAN_POINT ( 'NONE',  ( 3.999740995676851707, 47.42835276639851116, 4.270072082080261566 ) ) ;
#11006=AXIS2_PLACEMENT_3D ( 'NONE', #5920, #4575, #11566 ) ;
#11025=AXIS2_PLACEMENT_3D ( 'NONE', #167, #6524, #5441 ) ;
#11035=EDGE_CURVE ( 'NONE', #1857, #5669, #8320, .T. ) ;
#11106=AXIS2_PLACEMENT_3D ( 'NONE', #9992, #14460, #4453 ) ;
#11111=DIRECTION ( 'NONE',  ( 0.000000000000000000, 0.000000000000000000, 1.000000000000000000 ) ) ;
#11166=ADVANCED_BREP_SHAPE_REPRESENTATION ( '', ( #6873, #11025 ), #1200 ) ;
#11167=ORIENTED_EDGE ( 'NONE', *, *, #8195, .F. ) ;
#11241=EDGE_CURVE ( 'NONE', #14098, #9561, #1912, .T. ) ;
#11243=CARTESIAN_POINT ( 'NONE',  ( 8.000000000000000000, 40.49999999999999289, 0.000000000000000000 ) ) ;
#11248=AXIS2_PLACEMENT_3D ( 'NONE', #6134, #12800, #4119 ) ;
#11308=AXIS2_PLACEMENT_3D ( 'NONE', #3427, #13603, #7802 ) ;
#11336=ORIENTED_EDGE ( 'NONE', *, *, #1387, .T. ) ;
#11348=CYLINDRICAL_SURFACE ( 'NONE', #11006, 8.000000000000000000 ) ;
#11368=CARTESIAN_POINT ( 'NONE',  ( -8.000000000000000000, 25.49999999999996803, 0.000000000000000000 ) ) ;
#11389=AXIS2_PLACEMENT_3D ( 'NONE', #12538, #7473, #1724 ) ;
#11397=VECTOR ( 'NONE', #6687, 1000.000000000000000 ) ;
#11400=DIRECTION ( 'NONE',  ( 0.000000000000000000, 0.000000000000000000, 1.000000000000000000 ) ) ;
#11415=EDGE_CURVE ( 'NONE', #6358, #6826, #1010, .T. ) ;
#11437=ORIENTED_EDGE ( 'NONE', *, *, #4883, .T. ) ;
#11486=VERTEX_POINT ( 'NONE', #4330 ) ;
#11512=DIRECTION ( 'NONE',  ( 0.000000000000000000, 1.000000000000000000, 0.000000000000000000 ) ) ;
#11542=EDGE_CURVE ( 'NONE', #1857, #1693, #11700, .T. ) ;
#11550=CARTESIAN_POINT ( 'NONE',  ( 0.000000000000000000, 25.49999999999996803, 0.000000000000000000 ) ) ;
#11566=DIRECTION ( 'NONE',  ( -1.000000000000000000, 0.000000000000000000, 0.000000000000000000 ) ) ;
#11567=EDGE_CURVE ( 'NONE', #12253, #5260, #3584, .T. ) ;
#11593=CARTESIAN_POINT ( 'NONE',  ( 0.000000000000000000, 249.5765550933606391, 4.000000000000003553 ) ) ;
#11674=LINE ( 'NONE', #13890, #2426 ) ;
#11700=CIRCLE ( 'NONE', #13121, 8.000000000000000000 ) ;
#11716=AXIS2_PLACEMENT_3D ( 'NONE', #12456, #7455, #9371 ) ;
#11742=CARTESIAN_POINT ( 'NONE',  ( 0.000000000000000000, 249.5765550933606391, 4.000000000000003553 ) ) ;
#11775=ORIENTED_EDGE ( 'NONE', *, *, #11801, .T. ) ;
#11783=CARTESIAN_POINT ( 'NONE',  ( 2.018703368236236972, 48.24437551459758566, 7.463024472244906171 ) ) ;
#11800=ORIENTED_EDGE ( 'NONE', *, *, #2411, .T. ) ;
#11801=EDGE_CURVE ( 'NONE', #9561, #1257, #6902, .T. ) ;
#11837=PLANE ( 'NONE',  #188 ) ;
#11846=ORIENTED_EDGE ( 'NONE', *, *, #6614, .F. ) ;
#11852=CARTESIAN_POINT ( 'NONE',  ( 3.464648251117637301, 47.71258338693829160, 1.984273587230469982 ) ) ;
#11857=DIRECTION ( 'NONE',  ( 0.000000000000000000, 0.000000000000000000, -1.000000000000000000 ) ) ;
#11926=CARTESIAN_POINT ( 'NONE',  ( 3.868554393999077412, 47.50270580730570913, 5.050781263000352794 ) ) ;
#11929=PRODUCT_CONTEXT ( 'NONE', #7067, 'mechanical' ) ;
#11939=ORIENTED_EDGE ( 'NONE', *, *, #1387, .F. ) ;
#11977=DIRECTION ( 'NONE',  ( 0.000000000000000000, 0.000000000000000000, -1.000000000000000000 ) ) ;
#12061=CYLINDRICAL_SURFACE ( 'NONE', #10366, 2.750000000000003553 ) ;
#12074=ORIENTED_EDGE ( 'NONE', *, *, #2284, .F. ) ;
#12102=AXIS2_PLACEMENT_3D ( 'NONE', #1227, #8977, #2260 ) ;
#12151=ORIENTED_EDGE ( 'NONE', *, *, #8517, .T. ) ;
#12174=CIRCLE ( 'NONE', #5835, 4.000000000000000000 ) ;
#12181=AXIS2_PLACEMENT_3D ( 'NONE', #4118, #6053, #2866 ) ;
#12215=LINE ( 'NONE', #3511, #978 ) ;
#12249=SHAPE_REPRESENTATION_RELATIONSHIP ( 'NONE' , 'NONE' ,  #4432, #11166 ) ;
#12253=VERTEX_POINT ( 'NONE', #7231 ) ;
#12267=CARTESIAN_POINT ( 'NONE',  ( -8.000000000000000000, 40.49999999999999289, 0.000000000000000000 ) ) ;
#12349=DIRECTION ( 'NONE',  ( 0.000000000000000000, 0.000000000000000000, -1.000000000000000000 ) ) ;
#12407=DIRECTION ( 'NONE',  ( 0.000000000000000000, -1.000000000000000000, 0.000000000000000000 ) ) ;
#12424=MECHANICAL_DESIGN_GEOMETRIC_PRESENTATION_REPRESENTATION('',(#4269),#9375);
#12453=EDGE_CURVE ( 'NONE', #14098, #313, #12215, .T. ) ;
#12456=CARTESIAN_POINT ( 'NONE',  ( 0.000000000000000000, 25.49999999999996803, 8.000000000000007105 ) ) ;
#12457=( LENGTH_UNIT ( ) NAMED_UNIT ( * ) SI_UNIT ( .MILLI., .METRE. ) );
#12499=EDGE_CURVE ( 'NONE', #4722, #9673, #10222, .T. ) ;
#12521=FACE_OUTER_BOUND ( 'NONE', #1036, .T. ) ;
#12538=CARTESIAN_POINT ( 'NONE',  ( 0.000000000000000000, 249.5765550933606391, 4.000000000000003553 ) ) ;
#12548=CYLINDRICAL_SURFACE ( 'NONE', #11308, 2.750000000000003553 ) ;
#12567=EDGE_LOOP ( 'NONE', ( #13156, #13117, #13948, #8807 ) ) ;
#12569=FACE_OUTER_BOUND ( 'NONE', #9560, .T. ) ;
#12619=CARTESIAN_POINT ( 'NONE',  ( -1.790396195872466123, 48.30096731618026951, 7.586517658982195655 ) ) ;
#12778=CARTESIAN_POINT ( 'NONE',  ( 0.000000000000000000, 25.49999999999996803, 8.000000000000007105 ) ) ;
#12790=ORIENTED_EDGE ( 'NONE', *, *, #13492, .T. ) ;
#12800=DIRECTION ( 'NONE',  ( 0.000000000000000000, 0.000000000000000000, 1.000000000000000000 ) ) ;
#12855=CARTESIAN_POINT ( 'NONE',  ( -0.5330603548786400081, 48.48645934998780405, 7.973110123615588130 ) ) ;
#12883=SHAPE_DEFINITION_REPRESENTATION ( #10458, #4432 ) ;
#13015=CARTESIAN_POINT ( 'NONE',  ( -3.588625829919864341, 47.65084415347212854, 5.785846103500081661 ) ) ;
#13032=CARTESIAN_POINT ( 'NONE',  ( 3.588625829919864785, 47.65084415347212143, 5.785846103500077220 ) ) ;
#13046=DIRECTION ( 'NONE',  ( 0.000000000000000000, 0.000000000000000000, -1.000000000000000000 ) ) ;
#13063=EDGE_LOOP ( 'NONE', ( #13521, #8271, #7842, #8026 ) ) ;
#13089=CARTESIAN_POINT ( 'NONE',  ( 0.000000000000000000, 40.49999999999999289, 8.000000000000007105 ) ) ;
#13117=ORIENTED_EDGE ( 'NONE', *, *, #9460, .T. ) ;
#13121=AXIS2_PLACEMENT_3D ( 'NONE', #1441, #351, #13748 ) ;
#13124=CARTESIAN_POINT ( 'NONE',  ( 8.000000000000000000, 40.49999999999999289, 8.000000000000007105 ) ) ;
#13132=VECTOR ( 'NONE', #12407, 1000.000000000000000 ) ;
#13156=ORIENTED_EDGE ( 'NONE', *, *, #2411, .F. ) ;
#13159=CARTESIAN_POINT ( 'NONE',  ( -3.999740995676851707, 47.42835276639851116, 4.270072082080264231 ) ) ;
#13164=DIRECTION ( 'NONE',  ( 1.000000000000000000, 0.000000000000000000, 0.000000000000000000 ) ) ;
#13196=FACE_OUTER_BOUND ( 'NONE', #2229, .T. ) ;
#13208=CARTESIAN_POINT ( 'NONE',  ( -8.000000000000000000, 40.49999999999999289, 8.000000000000007105 ) ) ;
#13224=CARTESIAN_POINT ( 'NONE',  ( -3.177713737242648939, 47.84352126631786462, 6.443209146269483156 ) ) ;
#13241=CARTESIAN_POINT ( 'NONE',  ( 1.786241414228628255, 48.30187417244851389, 0.4115279878254324286 ) ) ;
#13281=EDGE_LOOP ( 'NONE', ( #2583, #6717, #14309, #9734 ) ) ;
#13291=ORIENTED_EDGE ( 'NONE', *, *, #2908, .T. ) ;
#13313=DIRECTION ( 'NONE',  ( 0.000000000000000000, -1.000000000000000000, 0.000000000000000000 ) ) ;
#13370=VECTOR ( 'NONE', #7227, 1000.000000000000000 ) ;
#13440=ORIENTED_EDGE ( 'NONE', *, *, #886, .F. ) ;
#13492=EDGE_CURVE ( 'NONE', #12253, #4722, #1465, .T. ) ;
#13521=ORIENTED_EDGE ( 'NONE', *, *, #7869, .T. ) ;
#13566=FACE_OUTER_BOUND ( 'NONE', #13281, .T. ) ;
#13567=FILL_AREA_STYLE ('',( #231 ) ) ;
#13598=ORIENTED_EDGE ( 'NONE', *, *, #11241, .T. ) ;
#13603=DIRECTION ( 'NONE',  ( 0.000000000000000000, 0.000000000000000000, -1.000000000000000000 ) ) ;
#13625=ORIENTED_EDGE ( 'NONE', *, *, #9460, .F. ) ;
#13702=ORIENTED_EDGE ( 'NONE', *, *, #1297, .F. ) ;
#13710=ORIENTED_EDGE ( 'NONE', *, *, #12453, .F. ) ;
#13712=DIRECTION ( 'NONE',  ( -1.000000000000000000, 0.000000000000000000, 0.000000000000000000 ) ) ;
#13741=CARTESIAN_POINT ( 'NONE',  ( -2.018703368236236084, 48.24437551459758566, 7.463024472244906171 ) ) ;
#13748=DIRECTION ( 'NONE',  ( 1.000000000000000000, 0.000000000000000000, 0.000000000000000000 ) ) ;
#13773=MECHANICAL_DESIGN_GEOMETRIC_PRESENTATION_REPRESENTATION('',(#10015),#3720);
#13792=UNCERTAINTY_MEASURE_WITH_UNIT (LENGTH_MEASURE( 1.000000000000000082E-05 ), #10331, 'distance_accuracy_value', 'NONE');
#13812=ORIENTED_EDGE ( 'NONE', *, *, #11035, .T. ) ;
#13826=DIRECTION ( 'NONE',  ( 0.000000000000000000, 0.000000000000000000, -1.000000000000000000 ) ) ;
#13837=PLANE ( 'NONE',  #6058 ) ;
#13890=CARTESIAN_POINT ( 'NONE',  ( 8.000000000000000000, 25.49999999999996803, 8.000000000000007105 ) ) ;
#13897=FACE_BOUND ( 'NONE', #1422, .T. ) ;
#13925=PLANE ( 'NONE',  #7533 ) ;
#13927=ORIENTED_EDGE ( 'NONE', *, *, #12453, .T. ) ;
#13948=ORIENTED_EDGE ( 'NONE', *, *, #886, .T. ) ;
#13961=( LENGTH_UNIT ( ) NAMED_UNIT ( * ) SI_UNIT ( .MILLI., .METRE. ) );
#13977=DIRECTION ( 'NONE',  ( 1.000000000000000000, 0.000000000000000000, 0.000000000000000000 ) ) ;
#14004=CARTESIAN_POINT ( 'NONE',  ( 0.000000000000000000, 25.49999999999996803, 8.000000000000007105 ) ) ;
#14041=CARTESIAN_POINT ( 'NONE',  ( -3.790690275325682812, 47.54583148236282142, 2.696316195168957819 ) ) ;
#14057=ORIENTED_EDGE ( 'NONE', *, *, #8517, .F. ) ;
#14058=ORIENTED_EDGE ( 'NONE', *, *, #7869, .F. ) ;
#14091=CARTESIAN_POINT ( 'NONE',  ( 0.000000000000000000, 25.49999999999996803, 0.000000000000000000 ) ) ;
#14098=VERTEX_POINT ( 'NONE', #1998 ) ;
#14113=CARTESIAN_POINT ( 'NONE',  ( -3.973244831464914029, 47.44383994248514824, 3.467973375954350068 ) ) ;
#14198=CARTESIAN_POINT ( 'NONE',  ( 3.868826622783372304, 47.50255440539075380, 2.950282236837604266 ) ) ;
#14265=DIRECTION ( 'NONE',  ( 0.000000000000000000, 0.000000000000000000, 1.000000000000000000 ) ) ;
#14267=CARTESIAN_POINT ( 'NONE',  ( 3.177713737242649827, 47.84352126631787172, 6.443209146269484933 ) ) ;
#14309=ORIENTED_EDGE ( 'NONE', *, *, #5526, .F. ) ;
#14339=CARTESIAN_POINT ( 'NONE',  ( 2.650472254991407706, 48.05066328782152141, 7.006789553262801284 ) ) ;
#14391=CIRCLE ( 'NONE', #827, 8.000000000000000000 ) ;
#14418=DIRECTION ( 'NONE',  ( 1.000000000000000000, 0.000000000000000000, 0.000000000000000000 ) ) ;
#14454=AXIS2_PLACEMENT_3D ( 'NONE', #235, #4580, #5776 ) ;
#14460=DIRECTION ( 'NONE',  ( 0.000000000000000000, 0.000000000000000000, 1.000000000000000000 ) ) ;
ENDSEC;
END-ISO-10303-21;
